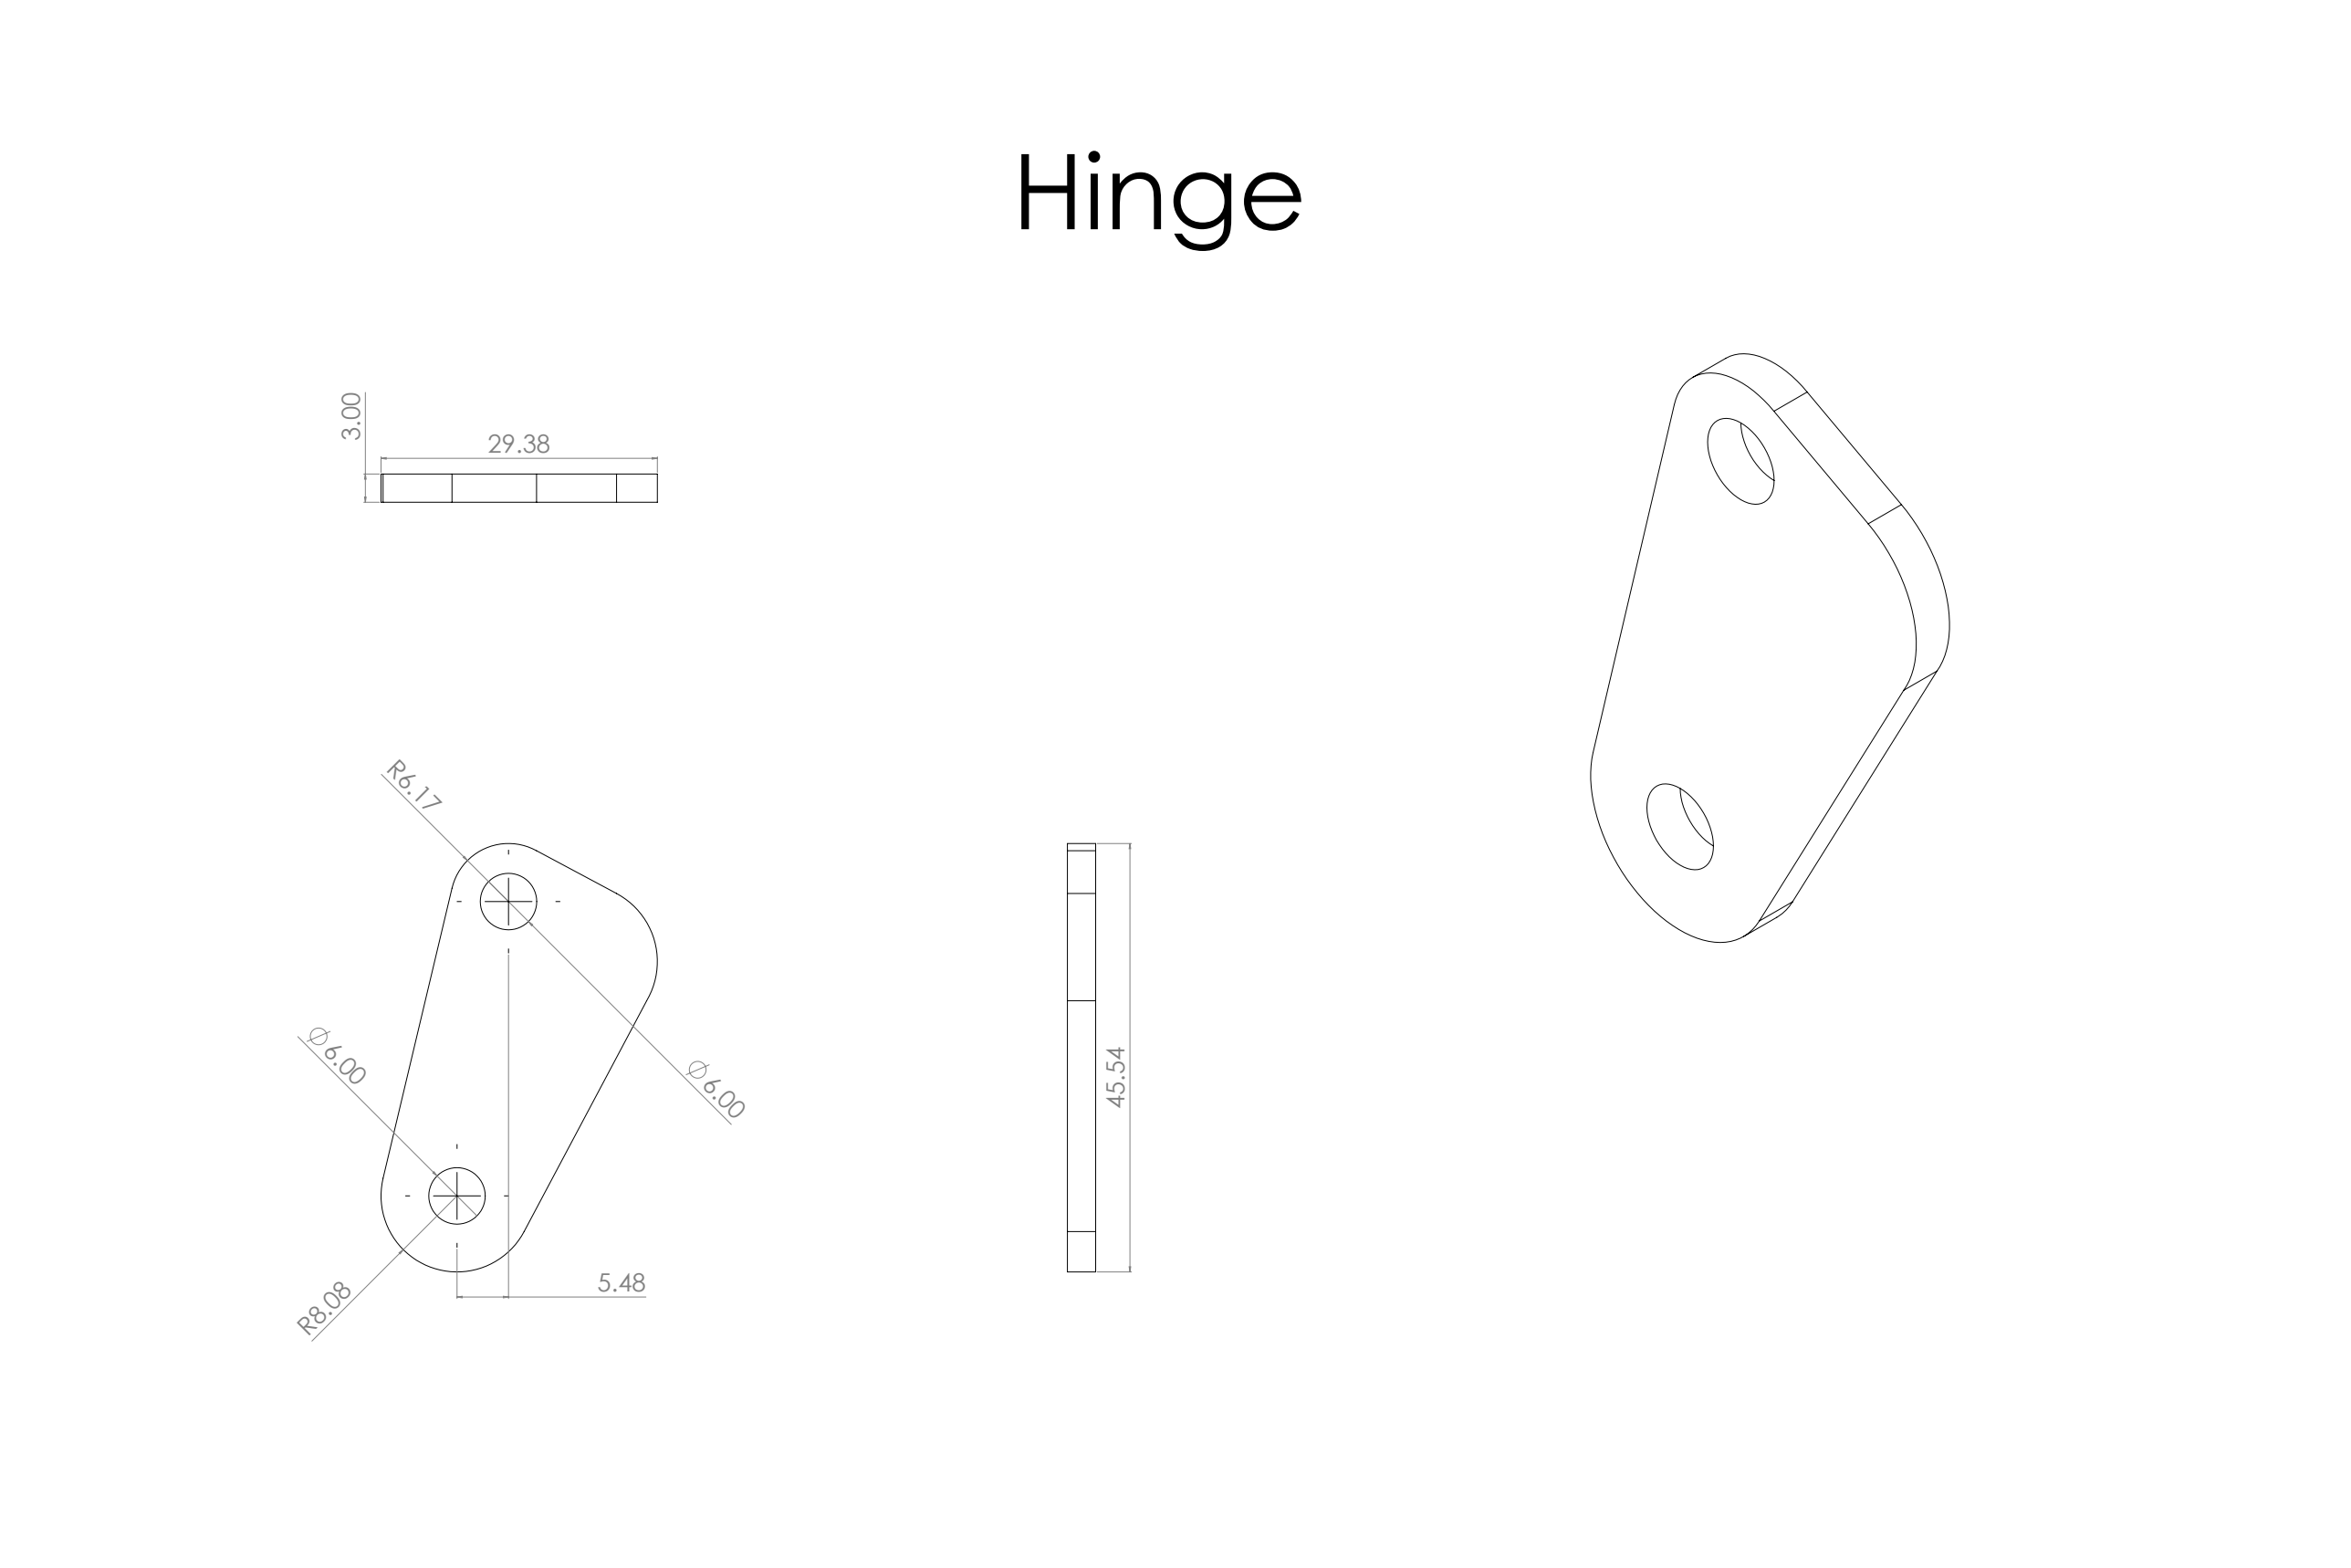
ISO-10303-21;
HEADER;
FILE_DESCRIPTION (('STEP AP214'),
    '1' );
FILE_NAME ('Hinge.step',
    '2026-10-24T22:54:28',
    ( '' ),
    ( '' ),
    'SwSTEP 2.0',
    'SolidWorks 2025',
    '' );
FILE_SCHEMA (( 'AUTOMOTIVE_DESIGN' ));
ENDSEC;

DATA;
#13=CARTESIAN_POINT ( 'NONE',  ( -63.96477757089261473, 34.57625524247897175, 12.50000000000000000 ) ) ;
#142=VERTEX_POINT ( 'NONE', #21892 ) ;
#147=CARTESIAN_POINT ( 'NONE',  ( -83.92837670882109080, 2.429809908903242555, 15.50000000000000000 ) ) ;
#153=VERTEX_POINT ( 'NONE', #35081 ) ;
#167=CIRCLE ( 'NONE', #21192, 3.000000000000002665 ) ;
#297=EDGE_CURVE ( 'NONE', #31547, #18087, #3886, .T. ) ;
#392=DIRECTION ( 'NONE',  ( -1.000000000000000000, 0.000000000000000000, 0.000000000000000000 ) ) ;
#485=FACE_OUTER_BOUND ( 'NONE', #18032, .T. ) ;
#713=VERTEX_POINT ( 'NONE', #13 ) ;
#743=CARTESIAN_POINT ( 'NONE',  ( -80.92837670882107659, 2.429809908903242555, 15.50000000000000000 ) ) ;
#852=DIRECTION ( 'NONE',  ( 1.000000000000000000, 0.000000000000000000, 0.000000000000000000 ) ) ;
#958=CARTESIAN_POINT ( 'NONE',  ( -75.45330471031414277, 33.71485196875532608, 15.50000000000000000 ) ) ;
#971=AXIS2_PLACEMENT_3D ( 'NONE', #36507, #21274, #21481 ) ;
#1225=FACE_OUTER_BOUND ( 'NONE', #8192, .T. ) ;
#1367=EDGE_CURVE ( 'NONE', #37942, #25139, #13140, .T. ) ;
#1424=ADVANCED_FACE ( 'NONE', ( #18777 ), #31557, .F. ) ;
#1458=ORIENTED_EDGE ( 'NONE', *, *, #11982, .T. ) ;
#1660=SHAPE_REPRESENTATION_RELATIONSHIP ( 'NONE' , 'NONE' ,  #29798, #21016 ) ;
#1742=ORIENTED_EDGE ( 'NONE', *, *, #27000, .F. ) ;
#1929=ORIENTED_EDGE ( 'NONE', *, *, #35756, .F. ) ;
#2065=CYLINDRICAL_SURFACE ( 'NONE', #35968, 8.080217238368769372 ) ;
#2190=DIRECTION ( 'NONE',  ( -1.000000000000000000, 0.000000000000000000, 0.000000000000000000 ) ) ;
#2205=EDGE_LOOP ( 'NONE', ( #36341, #27877, #24437, #30151 ) ) ;
#2358=AXIS2_PLACEMENT_3D ( 'NONE', #25493, #16604, #392 ) ;
#2457=EDGE_CURVE ( 'NONE', #4993, #21312, #12183, .T. ) ;
#2619=CARTESIAN_POINT ( 'NONE',  ( -77.92837670882107659, 2.429809908903242999, 12.50000000000000000 ) ) ;
#3062=ORIENTED_EDGE ( 'NONE', *, *, #33806, .T. ) ;
#3104=DIRECTION ( 'NONE',  ( 1.000000000000000000, 0.000000000000000000, -0.000000000000000000 ) ) ;
#3191=DIRECTION ( 'NONE',  ( 0.000000000000000000, 0.000000000000000000, 1.000000000000000000 ) ) ;
#3207=DIRECTION ( 'NONE',  ( -0.000000000000000000, -0.000000000000000000, -1.000000000000000000 ) ) ;
#3553=DIRECTION ( 'NONE',  ( 1.000000000000000000, 0.000000000000000000, 0.000000000000000000 ) ) ;
#3560=CARTESIAN_POINT ( 'NONE',  ( -72.46964309959683703, 39.11862660440054640, 12.50000000000000000 ) ) ;
#3575=DIRECTION ( 'NONE',  ( 0.000000000000000000, 0.000000000000000000, 1.000000000000000000 ) ) ;
#3746=ORIENTED_EDGE ( 'NONE', *, *, #21021, .F. ) ;
#3856=EDGE_CURVE ( 'NONE', #35794, #14683, #12318, .T. ) ;
#3886=CIRCLE ( 'NONE', #9103, 8.204531065793066347 ) ;
#3920=PLANE ( 'NONE',  #23999 ) ;
#4085=PLANE ( 'NONE',  #17432 ) ;
#4281=FACE_OUTER_BOUND ( 'NONE', #22061, .T. ) ;
#4356=ORIENTED_EDGE ( 'NONE', *, *, #3856, .T. ) ;
#4419=CIRCLE ( 'NONE', #38595, 3.000000000000002665 ) ;
#4709=EDGE_CURVE ( 'NONE', #37682, #713, #11903, .T. ) ;
#4778=AXIS2_PLACEMENT_3D ( 'NONE', #16988, #35159, #32068 ) ;
#4813=CIRCLE ( 'NONE', #4778, 3.000000000000002665 ) ;
#4993=VERTEX_POINT ( 'NONE', #27564 ) ;
#5090=ORIENTED_EDGE ( 'NONE', *, *, #27168, .T. ) ;
#5145=CARTESIAN_POINT ( 'NONE',  ( -60.75950795826495465, 23.17721540975219696, 15.50000000000000000 ) ) ;
#5228=LINE ( 'NONE', #35283, #20001 ) ;
#5260=DIRECTION ( 'NONE',  ( -0.000000000000000000, -0.000000000000000000, -1.000000000000000000 ) ) ;
#5338=DIRECTION ( 'NONE',  ( -0.000000000000000000, -0.000000000000000000, -1.000000000000000000 ) ) ;
#5585=DIRECTION ( 'NONE',  ( -0.8820753183692411348, 0.4711084086744811161, -0.000000000000000000 ) ) ;
#5689=ORIENTED_EDGE ( 'NONE', *, *, #37373, .T. ) ;
#5764=ORIENTED_EDGE ( 'NONE', *, *, #38341, .F. ) ;
#5839=CARTESIAN_POINT ( 'NONE',  ( -75.45330471031414277, 33.71485196875532608, 15.50000000000000000 ) ) ;
#5909=ORIENTED_EDGE ( 'NONE', *, *, #38341, .T. ) ;
#5971=DIRECTION ( 'NONE',  ( -0.000000000000000000, -0.000000000000000000, -1.000000000000000000 ) ) ;
#5993=DIRECTION ( 'NONE',  ( 0.000000000000000000, 0.000000000000000000, 1.000000000000000000 ) ) ;
#6108=LINE ( 'NONE', #147, #26129 ) ;
#6117=PRODUCT_DEFINITION_CONTEXT ( 'detailed design', #21603, 'design' ) ;
#6163=ORIENTED_EDGE ( 'NONE', *, *, #33342, .T. ) ;
#6165=ORIENTED_EDGE ( 'NONE', *, *, #30007, .F. ) ;
#6357=CARTESIAN_POINT ( 'NONE',  ( -72.46964309959683703, 39.11862660440054640, 15.50000000000000000 ) ) ;
#6573=ORIENTED_EDGE ( 'NONE', *, *, #1367, .T. ) ;
#6652=PLANE ( 'NONE',  #9688 ) ;
#6841=CARTESIAN_POINT ( 'NONE',  ( -75.45330471031414277, 33.71485196875532608, 15.50000000000000000 ) ) ;
#6847=EDGE_CURVE ( 'NONE', #8362, #37942, #24141, .T. ) ;
#6898=LINE ( 'NONE', #16549, #8340 ) ;
#7121=CARTESIAN_POINT ( 'NONE',  ( -73.79226524390077202, -1.360417495813321054, 12.50000000000000000 ) ) ;
#7198=CARTESIAN_POINT ( 'NONE',  ( -67.83000114521873058, 27.33924089054923101, 12.50000000000000000 ) ) ;
#7289=ORIENTED_EDGE ( 'NONE', *, *, #15777, .F. ) ;
#7353=CYLINDRICAL_SURFACE ( 'NONE', #2358, 8.204531065793066347 ) ;
#7446=VECTOR ( 'NONE', #15507, 1000.000000000000000 ) ;
#7615=EDGE_CURVE ( 'NONE', #4993, #32730, #11773, .T. ) ;
#7637=EDGE_LOOP ( 'NONE', ( #24808, #1742, #36801, #29004 ) ) ;
#7704=FACE_OUTER_BOUND ( 'NONE', #26436, .T. ) ;
#8006=AXIS2_PLACEMENT_3D ( 'NONE', #24944, #37477, #24523 ) ;
#8131=LINE ( 'NONE', #20702, #16745 ) ;
#8138=ORIENTED_EDGE ( 'NONE', *, *, #37421, .F. ) ;
#8192=EDGE_LOOP ( 'NONE', ( #31555, #7289, #3746, #23538 ) ) ;
#8202=ORIENTED_EDGE ( 'NONE', *, *, #20447, .F. ) ;
#8340=VECTOR ( 'NONE', #26043, 1000.000000000000000 ) ;
#8362=VERTEX_POINT ( 'NONE', #35558 ) ;
#8379=ORIENTED_EDGE ( 'NONE', *, *, #26172, .F. ) ;
#8548=CARTESIAN_POINT ( 'NONE',  ( -80.92837670882107659, 2.429809908903242555, 12.50000000000000000 ) ) ;
#8858=CARTESIAN_POINT ( 'NONE',  ( -72.46964309959683703, 39.11862660440054640, 12.50000000000000000 ) ) ;
#8979=UNCERTAINTY_MEASURE_WITH_UNIT (LENGTH_MEASURE( 1.000000000000000082E-05 ), #27662, 'distance_accuracy_value', 'NONE');
#9001=CIRCLE ( 'NONE', #27399, 6.172764123155108251 ) ;
#9103=AXIS2_PLACEMENT_3D ( 'NONE', #18793, #3191, #15707 ) ;
#9225=DIRECTION ( 'NONE',  ( -0.000000000000000000, -0.000000000000000000, -1.000000000000000000 ) ) ;
#9357=EDGE_LOOP ( 'NONE', ( #3062, #30595 ) ) ;
#9403=CARTESIAN_POINT ( 'NONE',  ( -60.75950795826495465, 23.17721540975219696, 15.50000000000000000 ) ) ;
#9485=DIRECTION ( 'NONE',  ( 0.000000000000000000, 0.000000000000000000, 1.000000000000000000 ) ) ;
#9608=LINE ( 'NONE', #13297, #29469 ) ;
#9659=CARTESIAN_POINT ( 'NONE',  ( -75.45330471031414277, 33.71485196875532608, 12.50000000000000000 ) ) ;
#9688=AXIS2_PLACEMENT_3D ( 'NONE', #38526, #19203, #22711 ) ;
#9744=AXIS2_PLACEMENT_3D ( 'NONE', #39630, #5260, #2190 ) ;
#9755=DIRECTION ( 'NONE',  ( 1.000000000000000000, 0.000000000000000000, 0.000000000000000000 ) ) ;
#9776=VECTOR ( 'NONE', #37121, 1000.000000000000000 ) ;
#9791=DIRECTION ( 'NONE',  ( 0.000000000000000000, 0.000000000000000000, 1.000000000000000000 ) ) ;
#10228=FACE_OUTER_BOUND ( 'NONE', #19075, .T. ) ;
#10926=LINE ( 'NONE', #23504, #25495 ) ;
#10980=DIRECTION ( 'NONE',  ( -0.4711084086744811716, -0.8820753183692411348, 0.000000000000000000 ) ) ;
#11093=VERTEX_POINT ( 'NONE', #14114 ) ;
#11196=CARTESIAN_POINT ( 'NONE',  ( -72.45330471031414277, 33.71485196875532608, 12.50000000000000000 ) ) ;
#11479=DIRECTION ( 'NONE',  ( 0.000000000000000000, 0.000000000000000000, 1.000000000000000000 ) ) ;
#11604=EDGE_CURVE ( 'NONE', #25139, #37682, #36716, .T. ) ;
#11674=ORIENTED_EDGE ( 'NONE', *, *, #21868, .F. ) ;
#11773=CIRCLE ( 'NONE', #34844, 3.000000000000002665 ) ;
#11903=CIRCLE ( 'NONE', #34972, 8.204531065793066347 ) ;
#11982=EDGE_CURVE ( 'NONE', #11093, #35794, #36088, .T. ) ;
#12000=( NAMED_UNIT ( * ) PLANE_ANGLE_UNIT ( ) SI_UNIT ( $, .RADIAN. ) );
#12083=EDGE_CURVE ( 'NONE', #713, #32955, #33606, .T. ) ;
#12183=LINE ( 'NONE', #37497, #38140 ) ;
#12318=LINE ( 'NONE', #37430, #40162 ) ;
#12344=ORIENTED_EDGE ( 'NONE', *, *, #6847, .T. ) ;
#12608=CARTESIAN_POINT ( 'NONE',  ( -81.45877670850643426, 35.14220020903839270, 15.50000000000000000 ) ) ;
#12625=ORIENTED_EDGE ( 'NONE', *, *, #11982, .F. ) ;
#12814=DIRECTION ( 'NONE',  ( 1.000000000000000000, 0.000000000000000000, 0.000000000000000000 ) ) ;
#12952=AXIS2_PLACEMENT_3D ( 'NONE', #25326, #40534, #40335 ) ;
#13140=CIRCLE ( 'NONE', #40078, 8.080217238368769372 ) ;
#13229=DIRECTION ( 'NONE',  ( -0.000000000000000000, -0.000000000000000000, -1.000000000000000000 ) ) ;
#13297=CARTESIAN_POINT ( 'NONE',  ( -88.78960668556791802, 4.298224710795182091, 12.50000000000000000 ) ) ;
#13409=CIRCLE ( 'NONE', #39047, 3.000000000000002665 ) ;
#13669=ADVANCED_FACE ( 'NONE', ( #4281 ), #7353, .T. ) ;
#13955=CIRCLE ( 'NONE', #8006, 8.080217238368769372 ) ;
#14114=CARTESIAN_POINT ( 'NONE',  ( -83.92837670882109080, 2.429809908903242555, 15.50000000000000000 ) ) ;
#14429=ADVANCED_FACE ( 'NONE', ( #10228, #35381, #19710 ), #4085, .F. ) ;
#14510=CYLINDRICAL_SURFACE ( 'NONE', #9744, 8.080217238368769372 ) ;
#14579=CARTESIAN_POINT ( 'NONE',  ( -80.92837670882107659, 2.429809908903242555, 15.50000000000000000 ) ) ;
#14614=AXIS2_PLACEMENT_3D ( 'NONE', #19027, #18403, #9755 ) ;
#14683=VERTEX_POINT ( 'NONE', #2619 ) ;
#14708=FACE_OUTER_BOUND ( 'NONE', #31494, .T. ) ;
#14728=ORIENTED_EDGE ( 'NONE', *, *, #20447, .T. ) ;
#14854=CARTESIAN_POINT ( 'NONE',  ( -72.45330471031414277, 33.71485196875532608, 15.50000000000000000 ) ) ;
#14979=CYLINDRICAL_SURFACE ( 'NONE', #29462, 3.000000000000002665 ) ;
#15106=ADVANCED_FACE ( 'NONE', ( #7704 ), #20254, .F. ) ;
#15260=LINE ( 'NONE', #34235, #32469 ) ;
#15313=CIRCLE ( 'NONE', #14614, 8.080217238368769372 ) ;
#15327=EDGE_CURVE ( 'NONE', #32730, #25213, #27653, .T. ) ;
#15492=DIRECTION ( 'NONE',  ( 0.000000000000000000, 0.000000000000000000, 1.000000000000000000 ) ) ;
#15507=DIRECTION ( 'NONE',  ( -0.000000000000000000, -0.000000000000000000, -1.000000000000000000 ) ) ;
#15694=DIRECTION ( 'NONE',  ( -0.000000000000000000, -0.000000000000000000, -1.000000000000000000 ) ) ;
#15707=DIRECTION ( 'NONE',  ( -1.000000000000000000, 0.000000000000000000, 0.000000000000000000 ) ) ;
#15715=CARTESIAN_POINT ( 'NONE',  ( -80.92837670882107659, 2.429809908903242555, 12.50000000000000000 ) ) ;
#15748=VERTEX_POINT ( 'NONE', #27294 ) ;
#15777=EDGE_CURVE ( 'NONE', #153, #15748, #15260, .T. ) ;
#15803=DIRECTION ( 'NONE',  ( -0.000000000000000000, -0.000000000000000000, -1.000000000000000000 ) ) ;
#15805=CARTESIAN_POINT ( 'NONE',  ( -72.46964309959683703, 39.11862660440054640, 15.50000000000000000 ) ) ;
#15916=CARTESIAN_POINT ( 'NONE',  ( -60.75950795826495465, 23.17721540975219696, 12.50000000000000000 ) ) ;
#15922=CARTESIAN_POINT ( 'NONE',  ( -75.45330471031414277, 33.71485196875532608, 15.50000000000000000 ) ) ;
#16024=CARTESIAN_POINT ( 'NONE',  ( -81.45877670850643426, 35.14220020903839270, 15.50000000000000000 ) ) ;
#16138=ORIENTED_EDGE ( 'NONE', *, *, #7615, .F. ) ;
#16230=ORIENTED_EDGE ( 'NONE', *, *, #11604, .F. ) ;
#16305=ADVANCED_FACE ( 'NONE', ( #19023 ), #34486, .F. ) ;
#16421=AXIS2_PLACEMENT_3D ( 'NONE', #6841, #15694, #28044 ) ;
#16549=CARTESIAN_POINT ( 'NONE',  ( -63.96477757089261473, 34.57625524247897175, 15.50000000000000000 ) ) ;
#16582=CARTESIAN_POINT ( 'NONE',  ( -72.46964309959683703, 39.11862660440054640, 15.50000000000000000 ) ) ;
#16604=DIRECTION ( 'NONE',  ( -0.000000000000000000, -0.000000000000000000, -1.000000000000000000 ) ) ;
#16613=VERTEX_POINT ( 'NONE', #27409 ) ;
#16745=VECTOR ( 'NONE', #39020, 1000.000000000000227 ) ;
#16810=ORIENTED_EDGE ( 'NONE', *, *, #37601, .F. ) ;
#16848=CARTESIAN_POINT ( 'NONE',  ( -75.45330471031414277, 33.71485196875532608, 12.50000000000000000 ) ) ;
#16902=AXIS2_PLACEMENT_3D ( 'NONE', #17724, #39354, #3104 ) ;
#16976=DIRECTION ( 'NONE',  ( -1.000000000000000000, 0.000000000000000000, 0.000000000000000000 ) ) ;
#16988=CARTESIAN_POINT ( 'NONE',  ( -80.92837670882107659, 2.429809908903242555, 12.50000000000000000 ) ) ;
#17048=ORIENTED_EDGE ( 'NONE', *, *, #12083, .F. ) ;
#17167=ADVANCED_FACE ( 'NONE', ( #1225 ), #3920, .F. ) ;
#17432=AXIS2_PLACEMENT_3D ( 'NONE', #8548, #20495, #30605 ) ;
#17491=PRODUCT_DEFINITION ( 'UNKNOWN', '', #34732, #6117 ) ;
#17528=AXIS2_PLACEMENT_3D ( 'NONE', #958, #35937, #16976 ) ;
#17724=CARTESIAN_POINT ( 'NONE',  ( -80.92837670882107659, 2.429809908903242555, 15.50000000000000000 ) ) ;
#17762=CARTESIAN_POINT ( 'NONE',  ( -60.75950795826495465, 23.17721540975219341, 12.50000000000000000 ) ) ;
#18032=EDGE_LOOP ( 'NONE', ( #19867, #8379, #37046, #39277 ) ) ;
#18086=ORIENTED_EDGE ( 'NONE', *, *, #20360, .F. ) ;
#18087=VERTEX_POINT ( 'NONE', #37947 ) ;
#18271=DIRECTION ( 'NONE',  ( 0.4690749385695654472, 0.8831583674551005680, -0.000000000000000000 ) ) ;
#18311=AXIS2_PLACEMENT_3D ( 'NONE', #743, #9791, #22371 ) ;
#18387=DIRECTION ( 'NONE',  ( 0.000000000000000000, 0.000000000000000000, 1.000000000000000000 ) ) ;
#18403=DIRECTION ( 'NONE',  ( 0.000000000000000000, 0.000000000000000000, 1.000000000000000000 ) ) ;
#18541=ORIENTED_EDGE ( 'NONE', *, *, #15327, .F. ) ;
#18777=FACE_OUTER_BOUND ( 'NONE', #2205, .T. ) ;
#18793=CARTESIAN_POINT ( 'NONE',  ( -67.83000114521873058, 27.33924089054923101, 15.50000000000000000 ) ) ;
#18904=DIRECTION ( 'NONE',  ( -0.8820753183692411348, 0.4711084086744811161, -0.000000000000000000 ) ) ;
#18931=DIRECTION ( 'NONE',  ( 1.000000000000000000, 0.000000000000000000, 0.000000000000000000 ) ) ;
#18936=CARTESIAN_POINT ( 'NONE',  ( -80.92837670882107659, 2.429809908903242555, 15.50000000000000000 ) ) ;
#18989=DIRECTION ( 'NONE',  ( -0.000000000000000000, -0.000000000000000000, -1.000000000000000000 ) ) ;
#19023=FACE_OUTER_BOUND ( 'NONE', #27109, .T. ) ;
#19027=CARTESIAN_POINT ( 'NONE',  ( -80.92837670882107659, 2.429809908903242555, 15.50000000000000000 ) ) ;
#19075=EDGE_LOOP ( 'NONE', ( #11674, #6165, #24930, #17048, #27279, #16230, #31180 ) ) ;
#19138=FACE_OUTER_BOUND ( 'NONE', #39548, .T. ) ;
#19156=CARTESIAN_POINT ( 'NONE',  ( -80.92837670882107659, 2.429809908903242555, 12.50000000000000000 ) ) ;
#19203=DIRECTION ( 'NONE',  ( -0.8831583674551005680, 0.4690749385695655027, 0.000000000000000000 ) ) ;
#19541=VECTOR ( 'NONE', #18904, 1000.000000000000000 ) ;
#19557=ORIENTED_EDGE ( 'NONE', *, *, #28469, .F. ) ;
#19710=FACE_BOUND ( 'NONE', #25573, .T. ) ;
#19867=ORIENTED_EDGE ( 'NONE', *, *, #11604, .T. ) ;
#19885=LINE ( 'NONE', #16582, #33742 ) ;
#20001=VECTOR ( 'NONE', #13229, 1000.000000000000000 ) ;
#20239=DIRECTION ( 'NONE',  ( -0.000000000000000000, -0.000000000000000000, -1.000000000000000000 ) ) ;
#20254=PLANE ( 'NONE',  #25881 ) ;
#20310=PRODUCT ( 'Hinge', 'Hinge', '', ( #20468 ) ) ;
#20360=EDGE_CURVE ( 'NONE', #32730, #4993, #37093, .T. ) ;
#20447=EDGE_CURVE ( 'NONE', #25213, #21312, #29234, .T. ) ;
#20453=CARTESIAN_POINT ( 'NONE',  ( -78.45330471031414277, 33.71485196875532608, 12.50000000000000000 ) ) ;
#20468=PRODUCT_CONTEXT ( 'NONE', #35030, 'mechanical' ) ;
#20495=DIRECTION ( 'NONE',  ( 0.000000000000000000, 0.000000000000000000, 1.000000000000000000 ) ) ;
#20642=ORIENTED_EDGE ( 'NONE', *, *, #21498, .F. ) ;
#20702=CARTESIAN_POINT ( 'NONE',  ( -88.78960668556791802, 4.298224710795182091, 15.50000000000000000 ) ) ;
#20812=CIRCLE ( 'NONE', #12952, 6.172764123155108251 ) ;
#21016=ADVANCED_BREP_SHAPE_REPRESENTATION ( '', ( #26623, #30744 ), #31385 ) ;
#21021=EDGE_CURVE ( 'NONE', #40083, #153, #8131, .T. ) ;
#21116=ORIENTED_EDGE ( 'NONE', *, *, #26172, .T. ) ;
#21192=AXIS2_PLACEMENT_3D ( 'NONE', #25960, #34841, #852 ) ;
#21258=ORIENTED_EDGE ( 'NONE', *, *, #32114, .T. ) ;
#21274=DIRECTION ( 'NONE',  ( 0.000000000000000000, 0.000000000000000000, 1.000000000000000000 ) ) ;
#21312=VERTEX_POINT ( 'NONE', #20453 ) ;
#21481=DIRECTION ( 'NONE',  ( 1.000000000000000000, 0.000000000000000000, 0.000000000000000000 ) ) ;
#21498=EDGE_CURVE ( 'NONE', #142, #25139, #5228, .T. ) ;
#21499=DIRECTION ( 'NONE',  ( 1.000000000000000000, 0.000000000000000000, 0.000000000000000000 ) ) ;
#21603=APPLICATION_CONTEXT ( 'automotive_design' ) ;
#21805=FACE_OUTER_BOUND ( 'NONE', #7637, .T. ) ;
#21825=DIRECTION ( 'NONE',  ( -1.000000000000000000, 0.000000000000000000, 0.000000000000000000 ) ) ;
#21857=DIRECTION ( 'NONE',  ( -0.000000000000000000, -0.000000000000000000, -1.000000000000000000 ) ) ;
#21868=EDGE_CURVE ( 'NONE', #15748, #37942, #26591, .T. ) ;
#21885=LINE ( 'NONE', #12608, #31305 ) ;
#21892=CARTESIAN_POINT ( 'NONE',  ( -73.79226524390077202, -1.360417495813321054, 15.50000000000000000 ) ) ;
#22061=EDGE_LOOP ( 'NONE', ( #33378, #19557, #26073, #21116 ) ) ;
#22103=DIRECTION ( 'NONE',  ( 0.000000000000000000, 0.000000000000000000, 1.000000000000000000 ) ) ;
#22266=DIRECTION ( 'NONE',  ( 1.000000000000000000, 0.000000000000000000, 0.000000000000000000 ) ) ;
#22371=DIRECTION ( 'NONE',  ( 1.000000000000000000, 0.000000000000000000, 0.000000000000000000 ) ) ;
#22530=DIRECTION ( 'NONE',  ( -1.000000000000000000, 0.000000000000000000, 0.000000000000000000 ) ) ;
#22711=DIRECTION ( 'NONE',  ( -0.4690749385695654472, -0.8831583674551004570, 0.000000000000000000 ) ) ;
#22782=SHAPE_DEFINITION_REPRESENTATION ( #28523, #29798 ) ;
#23257=DIRECTION ( 'NONE',  ( 0.000000000000000000, 0.000000000000000000, 1.000000000000000000 ) ) ;
#23368=CYLINDRICAL_SURFACE ( 'NONE', #17528, 6.172764123155108251 ) ;
#23504=CARTESIAN_POINT ( 'NONE',  ( -60.75950795826495465, 23.17721540975219341, 15.50000000000000000 ) ) ;
#23538=ORIENTED_EDGE ( 'NONE', *, *, #35756, .T. ) ;
#23547=CARTESIAN_POINT ( 'NONE',  ( -89.00859394718985129, 2.429809908903242555, 15.50000000000000000 ) ) ;
#23561=DIRECTION ( 'NONE',  ( 0.8820753183692410238, -0.4711084086744811161, 0.000000000000000000 ) ) ;
#23665=( NAMED_UNIT ( * ) PLANE_ANGLE_UNIT ( ) SI_UNIT ( $, .RADIAN. ) );
#23999=AXIS2_PLACEMENT_3D ( 'NONE', #26124, #32709, #26518 ) ;
#24044=CARTESIAN_POINT ( 'NONE',  ( -75.45330471031414277, 33.71485196875532608, 12.50000000000000000 ) ) ;
#24141=LINE ( 'NONE', #23547, #34127 ) ;
#24437=ORIENTED_EDGE ( 'NONE', *, *, #33342, .F. ) ;
#24523=DIRECTION ( 'NONE',  ( 1.000000000000000000, 0.000000000000000000, 0.000000000000000000 ) ) ;
#24808=ORIENTED_EDGE ( 'NONE', *, *, #6847, .F. ) ;
#24930=ORIENTED_EDGE ( 'NONE', *, *, #37373, .F. ) ;
#24944=CARTESIAN_POINT ( 'NONE',  ( -80.92837670882107659, 2.429809908903242555, 15.50000000000000000 ) ) ;
#25139=VERTEX_POINT ( 'NONE', #7121 ) ;
#25213=VERTEX_POINT ( 'NONE', #11196 ) ;
#25326=CARTESIAN_POINT ( 'NONE',  ( -75.45330471031414277, 33.71485196875532608, 15.50000000000000000 ) ) ;
#25381=DIRECTION ( 'NONE',  ( -0.000000000000000000, -0.000000000000000000, -1.000000000000000000 ) ) ;
#25397=EDGE_CURVE ( 'NONE', #8362, #142, #15313, .T. ) ;
#25493=CARTESIAN_POINT ( 'NONE',  ( -67.83000114521873058, 27.33924089054923101, 15.50000000000000000 ) ) ;
#25495=VECTOR ( 'NONE', #18271, 1000.000000000000000 ) ;
#25573=EDGE_LOOP ( 'NONE', ( #6163, #14728 ) ) ;
#25667=DIRECTION ( 'NONE',  ( -0.2312332387574689563, -0.9728983447892853853, -0.000000000000000000 ) ) ;
#25699=EDGE_LOOP ( 'NONE', ( #1458, #4356, #38604, #5764 ) ) ;
#25719=DIRECTION ( 'NONE',  ( 0.000000000000000000, 0.000000000000000000, 1.000000000000000000 ) ) ;
#25810=( GEOMETRIC_REPRESENTATION_CONTEXT ( 3 ) GLOBAL_UNCERTAINTY_ASSIGNED_CONTEXT ( ( #8979 ) ) GLOBAL_UNIT_ASSIGNED_CONTEXT ( ( #27662, #12000, #37131 ) ) REPRESENTATION_CONTEXT ( 'NONE', 'WORKASPACE' ) );
#25864=ORIENTED_EDGE ( 'NONE', *, *, #25397, .F. ) ;
#25881=AXIS2_PLACEMENT_3D ( 'NONE', #29729, #10980, #23561 ) ;
#25960=CARTESIAN_POINT ( 'NONE',  ( -80.92837670882107659, 2.429809908903242555, 15.50000000000000000 ) ) ;
#26043=DIRECTION ( 'NONE',  ( -0.000000000000000000, -0.000000000000000000, -1.000000000000000000 ) ) ;
#26073=ORIENTED_EDGE ( 'NONE', *, *, #297, .F. ) ;
#26117=ORIENTED_EDGE ( 'NONE', *, *, #37421, .T. ) ;
#26124=CARTESIAN_POINT ( 'NONE',  ( -88.78960668556791802, 4.298224710795182091, 15.50000000000000000 ) ) ;
#26129=VECTOR ( 'NONE', #38196, 1000.000000000000000 ) ;
#26172=EDGE_CURVE ( 'NONE', #31547, #37682, #39513, .T. ) ;
#26230=CLOSED_SHELL ( 'NONE', ( #1424, #31482, #31765, #38756, #14429, #27437, #29059, #13669, #15106, #40476, #17167, #37879, #16305 ) ) ;
#26372=( NAMED_UNIT ( * ) SI_UNIT ( $, .STERADIAN. ) SOLID_ANGLE_UNIT ( ) );
#26436=EDGE_LOOP ( 'NONE', ( #39075, #32501, #8138, #29527 ) ) ;
#26518=DIRECTION ( 'NONE',  ( 0.2312332387574689285, 0.9728983447892853853, 0.000000000000000000 ) ) ;
#26591=CIRCLE ( 'NONE', #29241, 8.080217238368769372 ) ;
#26623=MANIFOLD_SOLID_BREP ( 'Boss-Extrude4', #26230 ) ;
#27000=EDGE_CURVE ( 'NONE', #153, #8362, #13955, .T. ) ;
#27109=EDGE_LOOP ( 'NONE', ( #18541, #29255, #32947, #8202 ) ) ;
#27168=EDGE_CURVE ( 'NONE', #35794, #11093, #167, .T. ) ;
#27279=ORIENTED_EDGE ( 'NONE', *, *, #4709, .F. ) ;
#27294=CARTESIAN_POINT ( 'NONE',  ( -88.78960668556791802, 4.298224710795182091, 12.50000000000000000 ) ) ;
#27399=AXIS2_PLACEMENT_3D ( 'NONE', #24044, #11479, #30442 ) ;
#27409=CARTESIAN_POINT ( 'NONE',  ( -83.92837670882109080, 2.429809908903242555, 12.50000000000000000 ) ) ;
#27437=ADVANCED_FACE ( 'NONE', ( #21805 ), #2065, .T. ) ;
#27564=CARTESIAN_POINT ( 'NONE',  ( -78.45330471031414277, 33.71485196875532608, 15.50000000000000000 ) ) ;
#27653=LINE ( 'NONE', #31371, #7446 ) ;
#27662=( LENGTH_UNIT ( ) NAMED_UNIT ( * ) SI_UNIT ( .MILLI., .METRE. ) );
#27809=EDGE_LOOP ( 'NONE', ( #12625, #32363 ) ) ;
#27877=ORIENTED_EDGE ( 'NONE', *, *, #15327, .T. ) ;
#27958=VERTEX_POINT ( 'NONE', #15805 ) ;
#28044=DIRECTION ( 'NONE',  ( -1.000000000000000000, 0.000000000000000000, 0.000000000000000000 ) ) ;
#28246=DIRECTION ( 'NONE',  ( 1.000000000000000000, 0.000000000000000000, 0.000000000000000000 ) ) ;
#28469=EDGE_CURVE ( 'NONE', #18087, #713, #6898, .T. ) ;
#28523=PRODUCT_DEFINITION_SHAPE ( 'NONE', 'NONE',  #17491 ) ;
#28564=ORIENTED_EDGE ( 'NONE', *, *, #21021, .T. ) ;
#29004=ORIENTED_EDGE ( 'NONE', *, *, #21868, .T. ) ;
#29059=ADVANCED_FACE ( 'NONE', ( #485 ), #6652, .F. ) ;
#29160=MECHANICAL_DESIGN_GEOMETRIC_PRESENTATION_REPRESENTATION('',(#34437),#25810);
#29234=CIRCLE ( 'NONE', #29892, 3.000000000000002665 ) ;
#29241=AXIS2_PLACEMENT_3D ( 'NONE', #19156, #5993, #22266 ) ;
#29255=ORIENTED_EDGE ( 'NONE', *, *, #20360, .T. ) ;
#29462=AXIS2_PLACEMENT_3D ( 'NONE', #37810, #15803, #31661 ) ;
#29469=VECTOR ( 'NONE', #25667, 1000.000000000000227 ) ;
#29527=ORIENTED_EDGE ( 'NONE', *, *, #28469, .T. ) ;
#29729=CARTESIAN_POINT ( 'NONE',  ( -72.46964309959683703, 39.11862660440054640, 15.50000000000000000 ) ) ;
#29798=SHAPE_REPRESENTATION ( 'Hinge', ( #30744 ), #31385 ) ;
#29892=AXIS2_PLACEMENT_3D ( 'NONE', #16848, #15492, #34464 ) ;
#29897=FACE_BOUND ( 'NONE', #27809, .T. ) ;
#30007=EDGE_CURVE ( 'NONE', #35192, #15748, #9608, .T. ) ;
#30151=ORIENTED_EDGE ( 'NONE', *, *, #2457, .F. ) ;
#30442=DIRECTION ( 'NONE',  ( -1.000000000000000000, 0.000000000000000000, 0.000000000000000000 ) ) ;
#30595=ORIENTED_EDGE ( 'NONE', *, *, #37601, .T. ) ;
#30605=DIRECTION ( 'NONE',  ( 1.000000000000000000, 0.000000000000000000, -0.000000000000000000 ) ) ;
#30744=AXIS2_PLACEMENT_3D ( 'NONE', #35448, #9485, #3553 ) ;
#30950=ORIENTED_EDGE ( 'NONE', *, *, #27000, .T. ) ;
#31180=ORIENTED_EDGE ( 'NONE', *, *, #1367, .F. ) ;
#31305=VECTOR ( 'NONE', #25381, 1000.000000000000000 ) ;
#31371=CARTESIAN_POINT ( 'NONE',  ( -72.45330471031414277, 33.71485196875532608, 15.50000000000000000 ) ) ;
#31385=( GEOMETRIC_REPRESENTATION_CONTEXT ( 3 ) GLOBAL_UNCERTAINTY_ASSIGNED_CONTEXT ( ( #34545 ) ) GLOBAL_UNIT_ASSIGNED_CONTEXT ( ( #32553, #23665, #26372 ) ) REPRESENTATION_CONTEXT ( 'NONE', 'WORKASPACE' ) );
#31448=EDGE_LOOP ( 'NONE', ( #5689, #1929, #35949, #38599 ) ) ;
#31482=ADVANCED_FACE ( 'NONE', ( #36802 ), #14979, .F. ) ;
#31494=EDGE_LOOP ( 'NONE', ( #25864, #12344, #6573, #20642 ) ) ;
#31547=VERTEX_POINT ( 'NONE', #9403 ) ;
#31555=ORIENTED_EDGE ( 'NONE', *, *, #30007, .T. ) ;
#31557=CYLINDRICAL_SURFACE ( 'NONE', #16421, 3.000000000000002665 ) ;
#31661=DIRECTION ( 'NONE',  ( -1.000000000000000000, 0.000000000000000000, 0.000000000000000000 ) ) ;
#31765=ADVANCED_FACE ( 'NONE', ( #14708 ), #14510, .T. ) ;
#31882=LINE ( 'NONE', #6357, #19541 ) ;
#32068=DIRECTION ( 'NONE',  ( 1.000000000000000000, 0.000000000000000000, 0.000000000000000000 ) ) ;
#32114=EDGE_CURVE ( 'NONE', #142, #31547, #10926, .T. ) ;
#32363=ORIENTED_EDGE ( 'NONE', *, *, #27168, .F. ) ;
#32469=VECTOR ( 'NONE', #21857, 1000.000000000000000 ) ;
#32501=ORIENTED_EDGE ( 'NONE', *, *, #33763, .F. ) ;
#32553=( LENGTH_UNIT ( ) NAMED_UNIT ( * ) SI_UNIT ( .MILLI., .METRE. ) );
#32709=DIRECTION ( 'NONE',  ( 0.9728983447892854963, -0.2312332387574689563, 0.000000000000000000 ) ) ;
#32730=VERTEX_POINT ( 'NONE', #14854 ) ;
#32732=DIRECTION ( 'NONE',  ( -1.000000000000000000, 0.000000000000000000, 0.000000000000000000 ) ) ;
#32782=CARTESIAN_POINT ( 'NONE',  ( -77.92837670882107659, 2.429809908903242999, 15.50000000000000000 ) ) ;
#32947=ORIENTED_EDGE ( 'NONE', *, *, #2457, .T. ) ;
#32955=VERTEX_POINT ( 'NONE', #3560 ) ;
#33139=AXIS2_PLACEMENT_3D ( 'NONE', #15922, #3207, #22530 ) ;
#33342=EDGE_CURVE ( 'NONE', #21312, #25213, #13409, .T. ) ;
#33378=ORIENTED_EDGE ( 'NONE', *, *, #4709, .T. ) ;
#33606=LINE ( 'NONE', #8858, #34822 ) ;
#33742=VECTOR ( 'NONE', #35753, 1000.000000000000000 ) ;
#33763=EDGE_CURVE ( 'NONE', #27958, #32955, #19885, .T. ) ;
#33806=EDGE_CURVE ( 'NONE', #16613, #14683, #4813, .T. ) ;
#34018=AXIS2_PLACEMENT_3D ( 'NONE', #18936, #5971, #21825 ) ;
#34127=VECTOR ( 'NONE', #20239, 1000.000000000000000 ) ;
#34235=CARTESIAN_POINT ( 'NONE',  ( -88.78960668556791802, 4.298224710795182091, 15.50000000000000000 ) ) ;
#34369=ORIENTED_EDGE ( 'NONE', *, *, #25397, .T. ) ;
#34437=STYLED_ITEM('',(#40773),#26623);
#34464=DIRECTION ( 'NONE',  ( 1.000000000000000000, 0.000000000000000000, 0.000000000000000000 ) ) ;
#34486=CYLINDRICAL_SURFACE ( 'NONE', #33139, 3.000000000000002665 ) ;
#34545=UNCERTAINTY_MEASURE_WITH_UNIT (LENGTH_MEASURE( 1.000000000000000082E-05 ), #32553, 'distance_accuracy_value', 'NONE');
#34732=PRODUCT_DEFINITION_FORMATION_WITH_SPECIFIED_SOURCE ( 'ANY', '', #20310, .NOT_KNOWN. ) ;
#34815=CARTESIAN_POINT ( 'NONE',  ( -89.00859394718985129, 2.429809908903242555, 12.50000000000000000 ) ) ;
#34822=VECTOR ( 'NONE', #5585, 1000.000000000000000 ) ;
#34841=DIRECTION ( 'NONE',  ( 0.000000000000000000, 0.000000000000000000, 1.000000000000000000 ) ) ;
#34844=AXIS2_PLACEMENT_3D ( 'NONE', #5839, #22103, #12814 ) ;
#34972=AXIS2_PLACEMENT_3D ( 'NONE', #7198, #23257, #32732 ) ;
#35030=APPLICATION_CONTEXT ( 'automotive_design' ) ;
#35081=CARTESIAN_POINT ( 'NONE',  ( -88.78960668556791802, 4.298224710795182091, 15.50000000000000000 ) ) ;
#35159=DIRECTION ( 'NONE',  ( 0.000000000000000000, 0.000000000000000000, 1.000000000000000000 ) ) ;
#35192=VERTEX_POINT ( 'NONE', #37783 ) ;
#35283=CARTESIAN_POINT ( 'NONE',  ( -73.79226524390077202, -1.360417495813321054, 15.50000000000000000 ) ) ;
#35381=FACE_BOUND ( 'NONE', #9357, .T. ) ;
#35448=CARTESIAN_POINT ( 'NONE',  ( 0.000000000000000000, 0.000000000000000000, 0.000000000000000000 ) ) ;
#35558=CARTESIAN_POINT ( 'NONE',  ( -89.00859394718985129, 2.429809908903242555, 15.50000000000000000 ) ) ;
#35753=DIRECTION ( 'NONE',  ( -0.000000000000000000, -0.000000000000000000, -1.000000000000000000 ) ) ;
#35756=EDGE_CURVE ( 'NONE', #40083, #35192, #21885, .T. ) ;
#35794=VERTEX_POINT ( 'NONE', #32782 ) ;
#35937=DIRECTION ( 'NONE',  ( -0.000000000000000000, -0.000000000000000000, -1.000000000000000000 ) ) ;
#35949=ORIENTED_EDGE ( 'NONE', *, *, #37960, .F. ) ;
#35968=AXIS2_PLACEMENT_3D ( 'NONE', #14579, #5338, #39705 ) ;
#36015=ORIENTED_EDGE ( 'NONE', *, *, #297, .T. ) ;
#36088=CIRCLE ( 'NONE', #18311, 3.000000000000002665 ) ;
#36216=EDGE_LOOP ( 'NONE', ( #30950, #34369, #21258, #36015, #26117, #37950, #28564 ) ) ;
#36341=ORIENTED_EDGE ( 'NONE', *, *, #7615, .T. ) ;
#36355=VECTOR ( 'NONE', #39104, 1000.000000000000000 ) ;
#36507=CARTESIAN_POINT ( 'NONE',  ( -75.45330471031414277, 33.71485196875532608, 15.50000000000000000 ) ) ;
#36716=LINE ( 'NONE', #17762, #9776 ) ;
#36801=ORIENTED_EDGE ( 'NONE', *, *, #15777, .T. ) ;
#36802=FACE_OUTER_BOUND ( 'NONE', #25699, .T. ) ;
#37046=ORIENTED_EDGE ( 'NONE', *, *, #32114, .F. ) ;
#37093=CIRCLE ( 'NONE', #971, 3.000000000000002665 ) ;
#37121=DIRECTION ( 'NONE',  ( 0.4690749385695654472, 0.8831583674551005680, -0.000000000000000000 ) ) ;
#37131=( NAMED_UNIT ( * ) SI_UNIT ( $, .STERADIAN. ) SOLID_ANGLE_UNIT ( ) );
#37254=CYLINDRICAL_SURFACE ( 'NONE', #34018, 3.000000000000002665 ) ;
#37373=EDGE_CURVE ( 'NONE', #32955, #35192, #9001, .T. ) ;
#37421=EDGE_CURVE ( 'NONE', #18087, #27958, #31882, .T. ) ;
#37430=CARTESIAN_POINT ( 'NONE',  ( -77.92837670882107659, 2.429809908903242999, 15.50000000000000000 ) ) ;
#37477=DIRECTION ( 'NONE',  ( 0.000000000000000000, 0.000000000000000000, 1.000000000000000000 ) ) ;
#37497=CARTESIAN_POINT ( 'NONE',  ( -78.45330471031414277, 33.71485196875532608, 15.50000000000000000 ) ) ;
#37507=CARTESIAN_POINT ( 'NONE',  ( -80.92837670882107659, 2.429809908903242555, 12.50000000000000000 ) ) ;
#37601=EDGE_CURVE ( 'NONE', #14683, #16613, #4419, .T. ) ;
#37682=VERTEX_POINT ( 'NONE', #15916 ) ;
#37783=CARTESIAN_POINT ( 'NONE',  ( -81.45877670850643426, 35.14220020903839270, 12.50000000000000000 ) ) ;
#37810=CARTESIAN_POINT ( 'NONE',  ( -80.92837670882107659, 2.429809908903242555, 15.50000000000000000 ) ) ;
#37879=ADVANCED_FACE ( 'NONE', ( #19138 ), #37254, .F. ) ;
#37942=VERTEX_POINT ( 'NONE', #34815 ) ;
#37947=CARTESIAN_POINT ( 'NONE',  ( -63.96477757089261473, 34.57625524247897175, 15.50000000000000000 ) ) ;
#37950=ORIENTED_EDGE ( 'NONE', *, *, #37960, .T. ) ;
#37960=EDGE_CURVE ( 'NONE', #27958, #40083, #20812, .T. ) ;
#38140=VECTOR ( 'NONE', #18989, 1000.000000000000000 ) ;
#38196=DIRECTION ( 'NONE',  ( -0.000000000000000000, -0.000000000000000000, -1.000000000000000000 ) ) ;
#38341=EDGE_CURVE ( 'NONE', #11093, #16613, #6108, .T. ) ;
#38396=FACE_OUTER_BOUND ( 'NONE', #31448, .T. ) ;
#38526=CARTESIAN_POINT ( 'NONE',  ( -60.75950795826495465, 23.17721540975219341, 15.50000000000000000 ) ) ;
#38595=AXIS2_PLACEMENT_3D ( 'NONE', #15715, #18387, #21499 ) ;
#38599=ORIENTED_EDGE ( 'NONE', *, *, #33763, .T. ) ;
#38604=ORIENTED_EDGE ( 'NONE', *, *, #33806, .F. ) ;
#38756=ADVANCED_FACE ( 'NONE', ( #29897, #39975, #40720 ), #39558, .T. ) ;
#39020=DIRECTION ( 'NONE',  ( -0.2312332387574689563, -0.9728983447892853853, -0.000000000000000000 ) ) ;
#39047=AXIS2_PLACEMENT_3D ( 'NONE', #9659, #25719, #18931 ) ;
#39075=ORIENTED_EDGE ( 'NONE', *, *, #12083, .T. ) ;
#39104=DIRECTION ( 'NONE',  ( -0.000000000000000000, -0.000000000000000000, -1.000000000000000000 ) ) ;
#39147=ORIENTED_EDGE ( 'NONE', *, *, #3856, .F. ) ;
#39277=ORIENTED_EDGE ( 'NONE', *, *, #21498, .T. ) ;
#39354=DIRECTION ( 'NONE',  ( 0.000000000000000000, 0.000000000000000000, 1.000000000000000000 ) ) ;
#39513=LINE ( 'NONE', #5145, #36355 ) ;
#39548=EDGE_LOOP ( 'NONE', ( #39147, #5090, #5909, #16810 ) ) ;
#39558=PLANE ( 'NONE',  #16902 ) ;
#39577=EDGE_LOOP ( 'NONE', ( #16138, #18086 ) ) ;
#39630=CARTESIAN_POINT ( 'NONE',  ( -80.92837670882107659, 2.429809908903242555, 15.50000000000000000 ) ) ;
#39705=DIRECTION ( 'NONE',  ( -1.000000000000000000, 0.000000000000000000, 0.000000000000000000 ) ) ;
#39975=FACE_OUTER_BOUND ( 'NONE', #36216, .T. ) ;
#40078=AXIS2_PLACEMENT_3D ( 'NONE', #37507, #3575, #28246 ) ;
#40083=VERTEX_POINT ( 'NONE', #16024 ) ;
#40162=VECTOR ( 'NONE', #9225, 1000.000000000000000 ) ;
#40335=DIRECTION ( 'NONE',  ( -1.000000000000000000, 0.000000000000000000, 0.000000000000000000 ) ) ;
#40476=ADVANCED_FACE ( 'NONE', ( #38396 ), #23368, .T. ) ;
#40534=DIRECTION ( 'NONE',  ( 0.000000000000000000, 0.000000000000000000, 1.000000000000000000 ) ) ;
#40720=FACE_BOUND ( 'NONE', #39577, .T. ) ;
#40767=COLOUR_RGB('Off White',0.89,0.88,0.83);
#40768=FILL_AREA_STYLE_COLOUR('',#40767);
#40769=FILL_AREA_STYLE('',(#40768));
#40770=SURFACE_STYLE_FILL_AREA(#40769);
#40771=SURFACE_SIDE_STYLE('',(#40770));
#40772=SURFACE_STYLE_USAGE(.BOTH.,#40771);
#40773=PRESENTATION_STYLE_ASSIGNMENT((#40772));
ENDSEC;
END-ISO-10303-21;
